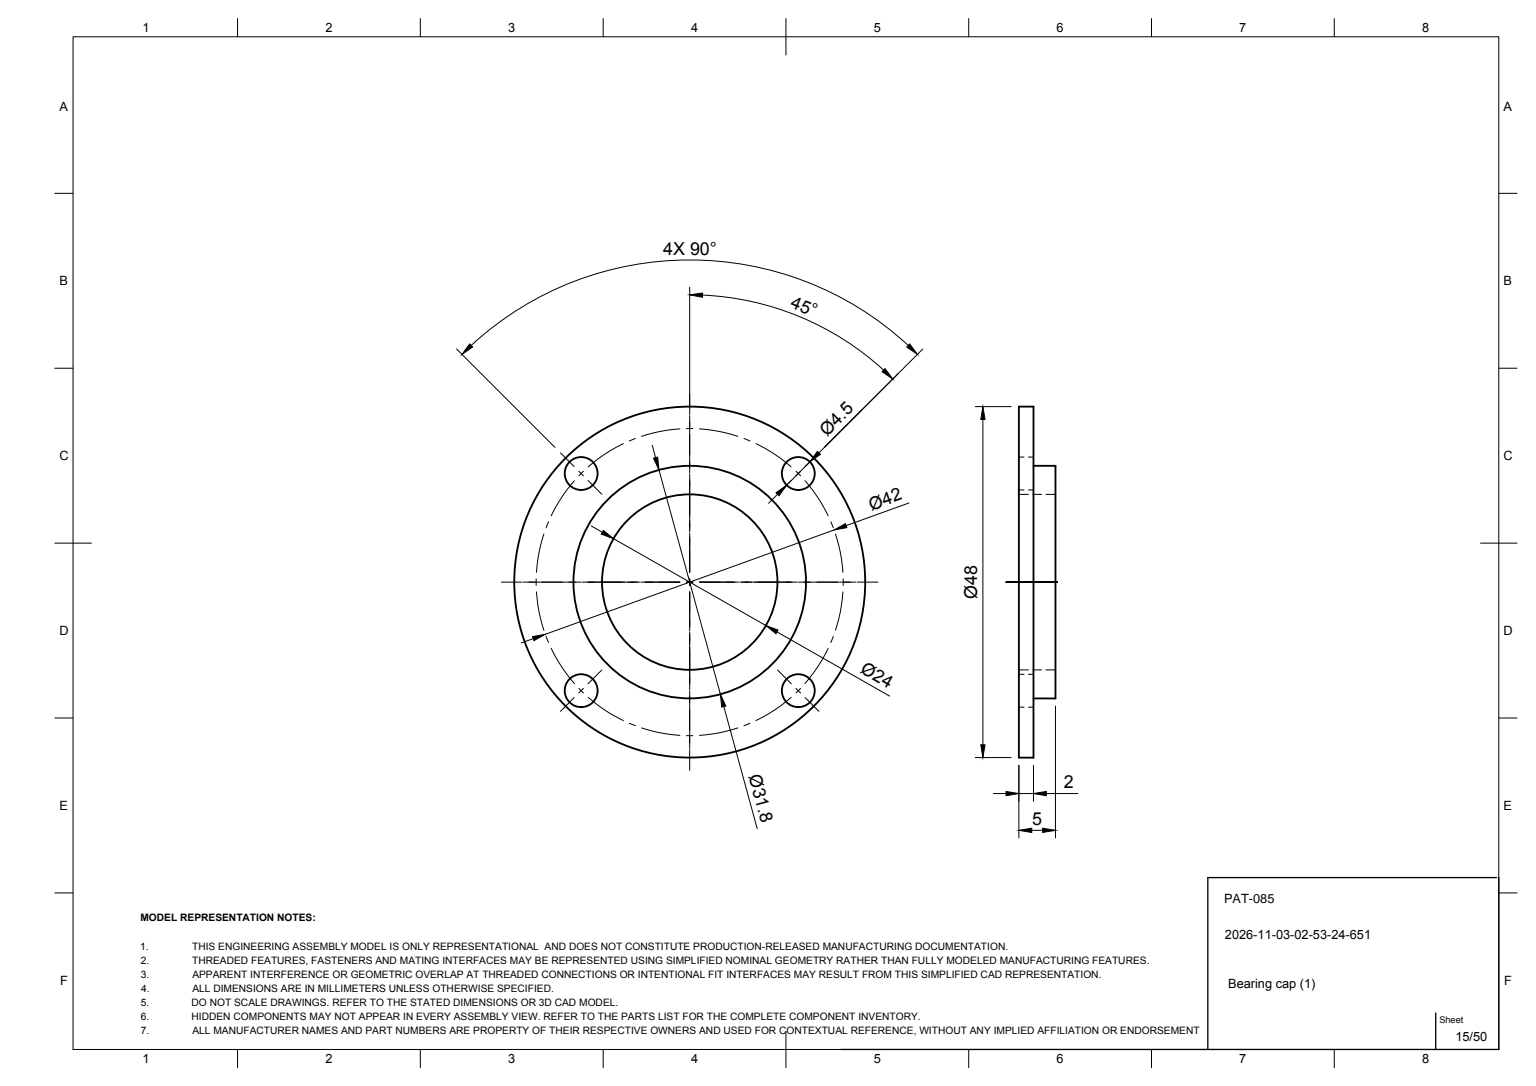
ISO-10303-21;
HEADER;
/* Generated by software containing ST-Developer
 * from STEP Tools, Inc. (www.steptools.com) 
 */

FILE_DESCRIPTION(
/* description */ ('Rack and pinion manual slide'),
/* implementation_level */ '2;1');

FILE_NAME(
/* name */ 'Bearing cap (1).step',
/* time_stamp */ '2026-10-28T03:22:49-07:00',
/* author */ (''),
/* organization */ (''),
/* preprocessor_version */ 'ST-DEVELOPER v20.2',
/* originating_system */ 'Autodesk Translation Framework v15.17.0.0',
/* authorisation */ '');

FILE_SCHEMA (('AUTOMOTIVE_DESIGN { 1 0 10303 214 3 1 1 }'));
ENDSEC;

DATA;
#10=MECHANICAL_DESIGN_GEOMETRIC_PRESENTATION_REPRESENTATION('',(#742),#34851);
#650=SHAPE_REPRESENTATION_RELATIONSHIP('SRR','None',#35085,#696);
#696=ADVANCED_BREP_SHAPE_REPRESENTATION('',(#795),#34810);
#742=STYLED_ITEM('',(#35411),#795);
#795=MANIFOLD_SOLID_BREP('Body1',#13762);
#910=FACE_BOUND('',#2464,.T.);
#911=FACE_BOUND('',#2468,.T.);
#912=FACE_BOUND('',#2469,.T.);
#913=FACE_BOUND('',#2470,.T.);
#914=FACE_BOUND('',#2471,.T.);
#915=FACE_BOUND('',#2472,.T.);
#916=FACE_BOUND('',#2474,.T.);
#917=FACE_BOUND('',#2475,.T.);
#918=FACE_BOUND('',#2476,.T.);
#919=FACE_BOUND('',#2477,.T.);
#920=FACE_BOUND('',#2478,.T.);
#1109=PLANE('',#14536);
#1110=PLANE('',#14543);
#1111=PLANE('',#14544);
#1642=FACE_OUTER_BOUND('',#2458,.T.);
#1643=FACE_OUTER_BOUND('',#2459,.T.);
#1644=FACE_OUTER_BOUND('',#2460,.T.);
#1645=FACE_OUTER_BOUND('',#2461,.T.);
#1646=FACE_OUTER_BOUND('',#2462,.T.);
#1647=FACE_OUTER_BOUND('',#2463,.T.);
#1648=FACE_OUTER_BOUND('',#2465,.T.);
#1649=FACE_OUTER_BOUND('',#2466,.T.);
#1650=FACE_OUTER_BOUND('',#2467,.T.);
#1651=FACE_OUTER_BOUND('',#2473,.T.);
#2458=EDGE_LOOP('',(#9726,#9727,#9728,#9729));
#2459=EDGE_LOOP('',(#9730,#9731,#9732,#9733));
#2460=EDGE_LOOP('',(#9734,#9735,#9736,#9737));
#2461=EDGE_LOOP('',(#9738,#9739,#9740,#9741));
#2462=EDGE_LOOP('',(#9742,#9743,#9744,#9745));
#2463=EDGE_LOOP('',(#9746));
#2464=EDGE_LOOP('',(#9747));
#2465=EDGE_LOOP('',(#9748,#9749,#9750,#9751));
#2466=EDGE_LOOP('',(#9752,#9753,#9754,#9755));
#2467=EDGE_LOOP('',(#9756));
#2468=EDGE_LOOP('',(#9757));
#2469=EDGE_LOOP('',(#9758));
#2470=EDGE_LOOP('',(#9759));
#2471=EDGE_LOOP('',(#9760));
#2472=EDGE_LOOP('',(#9761));
#2473=EDGE_LOOP('',(#9762));
#2474=EDGE_LOOP('',(#9763));
#2475=EDGE_LOOP('',(#9764));
#2476=EDGE_LOOP('',(#9765));
#2477=EDGE_LOOP('',(#9766));
#2478=EDGE_LOOP('',(#9767));
#3386=LINE('',#19991,#4677);
#3387=LINE('',#19997,#4678);
#3388=LINE('',#20003,#4679);
#3389=LINE('',#20009,#4680);
#3390=LINE('',#20015,#4681);
#3391=LINE('',#20023,#4682);
#3392=LINE('',#20028,#4683);
#4677=VECTOR('',#16174,0.225);
#4678=VECTOR('',#16181,0.225);
#4679=VECTOR('',#16188,0.225);
#4680=VECTOR('',#16195,0.225);
#4681=VECTOR('',#16202,1.59);
#4682=VECTOR('',#16213,1.2);
#4683=VECTOR('',#16218,2.4);
#5890=CIRCLE('',#14522,0.225);
#5891=CIRCLE('',#14523,0.225);
#5892=CIRCLE('',#14525,0.225);
#5893=CIRCLE('',#14526,0.225);
#5894=CIRCLE('',#14528,0.225);
#5895=CIRCLE('',#14529,0.225);
#5896=CIRCLE('',#14531,0.225);
#5897=CIRCLE('',#14532,0.225);
#5898=CIRCLE('',#14534,1.59);
#5899=CIRCLE('',#14535,1.59);
#5900=CIRCLE('',#14537,1.2);
#5901=CIRCLE('',#14539,1.2);
#5902=CIRCLE('',#14541,2.4);
#5903=CIRCLE('',#14542,2.4);
#6388=VERTEX_POINT('',#19988);
#6389=VERTEX_POINT('',#19990);
#6390=VERTEX_POINT('',#19994);
#6391=VERTEX_POINT('',#19996);
#6392=VERTEX_POINT('',#20000);
#6393=VERTEX_POINT('',#20002);
#6394=VERTEX_POINT('',#20006);
#6395=VERTEX_POINT('',#20008);
#6396=VERTEX_POINT('',#20012);
#6397=VERTEX_POINT('',#20014);
#6398=VERTEX_POINT('',#20018);
#6399=VERTEX_POINT('',#20021);
#6400=VERTEX_POINT('',#20025);
#6401=VERTEX_POINT('',#20027);
#7675=EDGE_CURVE('',#6388,#6388,#5890,.T.);
#7676=EDGE_CURVE('',#6388,#6389,#3386,.T.);
#7677=EDGE_CURVE('',#6389,#6389,#5891,.T.);
#7678=EDGE_CURVE('',#6390,#6390,#5892,.T.);
#7679=EDGE_CURVE('',#6390,#6391,#3387,.T.);
#7680=EDGE_CURVE('',#6391,#6391,#5893,.T.);
#7681=EDGE_CURVE('',#6392,#6392,#5894,.T.);
#7682=EDGE_CURVE('',#6392,#6393,#3388,.T.);
#7683=EDGE_CURVE('',#6393,#6393,#5895,.T.);
#7684=EDGE_CURVE('',#6394,#6394,#5896,.T.);
#7685=EDGE_CURVE('',#6394,#6395,#3389,.T.);
#7686=EDGE_CURVE('',#6395,#6395,#5897,.T.);
#7687=EDGE_CURVE('',#6396,#6396,#5898,.T.);
#7688=EDGE_CURVE('',#6396,#6397,#3390,.T.);
#7689=EDGE_CURVE('',#6397,#6397,#5899,.T.);
#7690=EDGE_CURVE('',#6398,#6398,#5900,.T.);
#7691=EDGE_CURVE('',#6399,#6399,#5901,.T.);
#7692=EDGE_CURVE('',#6399,#6398,#3391,.T.);
#7693=EDGE_CURVE('',#6400,#6400,#5902,.T.);
#7694=EDGE_CURVE('',#6400,#6401,#3392,.T.);
#7695=EDGE_CURVE('',#6401,#6401,#5903,.T.);
#9726=ORIENTED_EDGE('',*,*,#7675,.F.);
#9727=ORIENTED_EDGE('',*,*,#7676,.T.);
#9728=ORIENTED_EDGE('',*,*,#7677,.F.);
#9729=ORIENTED_EDGE('',*,*,#7676,.F.);
#9730=ORIENTED_EDGE('',*,*,#7678,.F.);
#9731=ORIENTED_EDGE('',*,*,#7679,.T.);
#9732=ORIENTED_EDGE('',*,*,#7680,.F.);
#9733=ORIENTED_EDGE('',*,*,#7679,.F.);
#9734=ORIENTED_EDGE('',*,*,#7681,.F.);
#9735=ORIENTED_EDGE('',*,*,#7682,.T.);
#9736=ORIENTED_EDGE('',*,*,#7683,.F.);
#9737=ORIENTED_EDGE('',*,*,#7682,.F.);
#9738=ORIENTED_EDGE('',*,*,#7684,.F.);
#9739=ORIENTED_EDGE('',*,*,#7685,.T.);
#9740=ORIENTED_EDGE('',*,*,#7686,.F.);
#9741=ORIENTED_EDGE('',*,*,#7685,.F.);
#9742=ORIENTED_EDGE('',*,*,#7687,.F.);
#9743=ORIENTED_EDGE('',*,*,#7688,.T.);
#9744=ORIENTED_EDGE('',*,*,#7689,.T.);
#9745=ORIENTED_EDGE('',*,*,#7688,.F.);
#9746=ORIENTED_EDGE('',*,*,#7689,.F.);
#9747=ORIENTED_EDGE('',*,*,#7690,.F.);
#9748=ORIENTED_EDGE('',*,*,#7691,.F.);
#9749=ORIENTED_EDGE('',*,*,#7692,.T.);
#9750=ORIENTED_EDGE('',*,*,#7690,.T.);
#9751=ORIENTED_EDGE('',*,*,#7692,.F.);
#9752=ORIENTED_EDGE('',*,*,#7693,.F.);
#9753=ORIENTED_EDGE('',*,*,#7694,.T.);
#9754=ORIENTED_EDGE('',*,*,#7695,.T.);
#9755=ORIENTED_EDGE('',*,*,#7694,.F.);
#9756=ORIENTED_EDGE('',*,*,#7693,.T.);
#9757=ORIENTED_EDGE('',*,*,#7691,.T.);
#9758=ORIENTED_EDGE('',*,*,#7686,.T.);
#9759=ORIENTED_EDGE('',*,*,#7683,.T.);
#9760=ORIENTED_EDGE('',*,*,#7680,.T.);
#9761=ORIENTED_EDGE('',*,*,#7677,.T.);
#9762=ORIENTED_EDGE('',*,*,#7695,.F.);
#9763=ORIENTED_EDGE('',*,*,#7687,.T.);
#9764=ORIENTED_EDGE('',*,*,#7684,.T.);
#9765=ORIENTED_EDGE('',*,*,#7681,.T.);
#9766=ORIENTED_EDGE('',*,*,#7678,.T.);
#9767=ORIENTED_EDGE('',*,*,#7675,.T.);
#12886=CYLINDRICAL_SURFACE('',#14521,0.225);
#12887=CYLINDRICAL_SURFACE('',#14524,0.225);
#12888=CYLINDRICAL_SURFACE('',#14527,0.225);
#12889=CYLINDRICAL_SURFACE('',#14530,0.225);
#12890=CYLINDRICAL_SURFACE('',#14533,1.59);
#12891=CYLINDRICAL_SURFACE('',#14538,1.2);
#12892=CYLINDRICAL_SURFACE('',#14540,2.4);
#13120=ADVANCED_FACE('',(#1642),#12886,.F.);
#13121=ADVANCED_FACE('',(#1643),#12887,.F.);
#13122=ADVANCED_FACE('',(#1644),#12888,.F.);
#13123=ADVANCED_FACE('',(#1645),#12889,.F.);
#13124=ADVANCED_FACE('',(#1646),#12890,.T.);
#13125=ADVANCED_FACE('',(#1647,#910),#1109,.F.);
#13126=ADVANCED_FACE('',(#1648),#12891,.F.);
#13127=ADVANCED_FACE('',(#1649),#12892,.T.);
#13128=ADVANCED_FACE('',(#1650,#911,#912,#913,#914,#915),#1110,.T.);
#13129=ADVANCED_FACE('',(#1651,#916,#917,#918,#919,#920),#1111,.F.);
#13762=CLOSED_SHELL('',(#13120,#13121,#13122,#13123,#13124,#13125,#13126,
#13127,#13128,#13129));
#14520=AXIS2_PLACEMENT_3D('',#19986,#16168,#16169);
#14521=AXIS2_PLACEMENT_3D('',#19987,#16170,#16171);
#14522=AXIS2_PLACEMENT_3D('',#19989,#16172,#16173);
#14523=AXIS2_PLACEMENT_3D('',#19992,#16175,#16176);
#14524=AXIS2_PLACEMENT_3D('',#19993,#16177,#16178);
#14525=AXIS2_PLACEMENT_3D('',#19995,#16179,#16180);
#14526=AXIS2_PLACEMENT_3D('',#19998,#16182,#16183);
#14527=AXIS2_PLACEMENT_3D('',#19999,#16184,#16185);
#14528=AXIS2_PLACEMENT_3D('',#20001,#16186,#16187);
#14529=AXIS2_PLACEMENT_3D('',#20004,#16189,#16190);
#14530=AXIS2_PLACEMENT_3D('',#20005,#16191,#16192);
#14531=AXIS2_PLACEMENT_3D('',#20007,#16193,#16194);
#14532=AXIS2_PLACEMENT_3D('',#20010,#16196,#16197);
#14533=AXIS2_PLACEMENT_3D('',#20011,#16198,#16199);
#14534=AXIS2_PLACEMENT_3D('',#20013,#16200,#16201);
#14535=AXIS2_PLACEMENT_3D('',#20016,#16203,#16204);
#14536=AXIS2_PLACEMENT_3D('',#20017,#16205,#16206);
#14537=AXIS2_PLACEMENT_3D('',#20019,#16207,#16208);
#14538=AXIS2_PLACEMENT_3D('',#20020,#16209,#16210);
#14539=AXIS2_PLACEMENT_3D('',#20022,#16211,#16212);
#14540=AXIS2_PLACEMENT_3D('',#20024,#16214,#16215);
#14541=AXIS2_PLACEMENT_3D('',#20026,#16216,#16217);
#14542=AXIS2_PLACEMENT_3D('',#20029,#16219,#16220);
#14543=AXIS2_PLACEMENT_3D('',#20030,#16221,#16222);
#14544=AXIS2_PLACEMENT_3D('',#20031,#16223,#16224);
#16168=DIRECTION('axis',(0.,0.,1.));
#16169=DIRECTION('refdir',(1.,0.,0.));
#16170=DIRECTION('center_axis',(0.,1.,0.));
#16171=DIRECTION('ref_axis',(1.,0.,0.));
#16172=DIRECTION('center_axis',(0.,1.,0.));
#16173=DIRECTION('ref_axis',(1.,0.,0.));
#16174=DIRECTION('',(0.,1.,0.));
#16175=DIRECTION('center_axis',(0.,-1.,0.));
#16176=DIRECTION('ref_axis',(1.,0.,0.));
#16177=DIRECTION('center_axis',(0.,1.,0.));
#16178=DIRECTION('ref_axis',(1.,0.,0.));
#16179=DIRECTION('center_axis',(0.,1.,0.));
#16180=DIRECTION('ref_axis',(1.,0.,0.));
#16181=DIRECTION('',(0.,1.,0.));
#16182=DIRECTION('center_axis',(0.,-1.,0.));
#16183=DIRECTION('ref_axis',(1.,0.,0.));
#16184=DIRECTION('center_axis',(0.,1.,0.));
#16185=DIRECTION('ref_axis',(1.,0.,0.));
#16186=DIRECTION('center_axis',(0.,1.,0.));
#16187=DIRECTION('ref_axis',(1.,0.,0.));
#16188=DIRECTION('',(0.,1.,0.));
#16189=DIRECTION('center_axis',(0.,-1.,0.));
#16190=DIRECTION('ref_axis',(1.,0.,0.));
#16191=DIRECTION('center_axis',(0.,1.,0.));
#16192=DIRECTION('ref_axis',(1.,0.,0.));
#16193=DIRECTION('center_axis',(0.,1.,0.));
#16194=DIRECTION('ref_axis',(1.,0.,0.));
#16195=DIRECTION('',(0.,1.,0.));
#16196=DIRECTION('center_axis',(0.,-1.,0.));
#16197=DIRECTION('ref_axis',(1.,0.,0.));
#16198=DIRECTION('center_axis',(0.,1.,0.));
#16199=DIRECTION('ref_axis',(1.,0.,0.));
#16200=DIRECTION('center_axis',(0.,1.,0.));
#16201=DIRECTION('ref_axis',(1.,0.,0.));
#16202=DIRECTION('',(0.,-1.,0.));
#16203=DIRECTION('center_axis',(0.,1.,0.));
#16204=DIRECTION('ref_axis',(1.,0.,0.));
#16205=DIRECTION('center_axis',(0.,1.,0.));
#16206=DIRECTION('ref_axis',(1.,0.,0.));
#16207=DIRECTION('center_axis',(0.,-1.,0.));
#16208=DIRECTION('ref_axis',(1.,0.,0.));
#16209=DIRECTION('center_axis',(0.,1.,0.));
#16210=DIRECTION('ref_axis',(1.,0.,0.));
#16211=DIRECTION('center_axis',(0.,-1.,0.));
#16212=DIRECTION('ref_axis',(1.,0.,0.));
#16213=DIRECTION('',(0.,-1.,0.));
#16214=DIRECTION('center_axis',(0.,1.,0.));
#16215=DIRECTION('ref_axis',(1.,0.,0.));
#16216=DIRECTION('center_axis',(0.,1.,0.));
#16217=DIRECTION('ref_axis',(1.,0.,0.));
#16218=DIRECTION('',(0.,-1.,0.));
#16219=DIRECTION('center_axis',(0.,1.,0.));
#16220=DIRECTION('ref_axis',(1.,0.,0.));
#16221=DIRECTION('center_axis',(0.,1.,0.));
#16222=DIRECTION('ref_axis',(1.,0.,0.));
#16223=DIRECTION('center_axis',(0.,1.,0.));
#16224=DIRECTION('ref_axis',(1.,0.,0.));
#19986=CARTESIAN_POINT('',(0.,0.,0.));
#19987=CARTESIAN_POINT('Origin',(9.51507575950825,-3.5,8.76507575950825));
#19988=CARTESIAN_POINT('',(9.29007575950825,-3.4,8.76507575950825));
#19989=CARTESIAN_POINT('Origin',(9.51507575950825,-3.4,8.76507575950825));
#19990=CARTESIAN_POINT('',(9.29007575950825,-3.2,8.76507575950825));
#19991=CARTESIAN_POINT('',(9.29007575950825,-3.5,8.76507575950825));
#19992=CARTESIAN_POINT('Origin',(9.51507575950825,-3.2,8.76507575950825));
#19993=CARTESIAN_POINT('Origin',(9.51507575950825,-3.5,11.7349242404918));
#19994=CARTESIAN_POINT('',(9.29007575950825,-3.4,11.7349242404918));
#19995=CARTESIAN_POINT('Origin',(9.51507575950825,-3.4,11.7349242404918));
#19996=CARTESIAN_POINT('',(9.29007575950825,-3.2,11.7349242404918));
#19997=CARTESIAN_POINT('',(9.29007575950825,-3.5,11.7349242404918));
#19998=CARTESIAN_POINT('Origin',(9.51507575950825,-3.2,11.7349242404918));
#19999=CARTESIAN_POINT('Origin',(12.4849242404918,-3.5,11.7349242404918));
#20000=CARTESIAN_POINT('',(12.2599242404918,-3.4,11.7349242404918));
#20001=CARTESIAN_POINT('Origin',(12.4849242404918,-3.4,11.7349242404918));
#20002=CARTESIAN_POINT('',(12.2599242404918,-3.2,11.7349242404918));
#20003=CARTESIAN_POINT('',(12.2599242404918,-3.5,11.7349242404918));
#20004=CARTESIAN_POINT('Origin',(12.4849242404918,-3.2,11.7349242404918));
#20005=CARTESIAN_POINT('Origin',(12.4849242404917,-3.5,8.76507575950825));
#20006=CARTESIAN_POINT('',(12.2599242404917,-3.4,8.76507575950825));
#20007=CARTESIAN_POINT('Origin',(12.4849242404917,-3.4,8.76507575950825));
#20008=CARTESIAN_POINT('',(12.2599242404917,-3.2,8.76507575950825));
#20009=CARTESIAN_POINT('',(12.2599242404917,-3.5,8.76507575950825));
#20010=CARTESIAN_POINT('Origin',(12.4849242404917,-3.2,8.76507575950825));
#20011=CARTESIAN_POINT('Origin',(11.,-3.7,10.25));
#20012=CARTESIAN_POINT('',(9.41,-3.4,10.25));
#20013=CARTESIAN_POINT('Origin',(11.,-3.4,10.25));
#20014=CARTESIAN_POINT('',(9.41,-3.7,10.25));
#20015=CARTESIAN_POINT('',(9.41,-3.7,10.25));
#20016=CARTESIAN_POINT('Origin',(11.,-3.7,10.25));
#20017=CARTESIAN_POINT('Origin',(11.,-3.7,10.25));
#20018=CARTESIAN_POINT('',(9.8,-3.7,10.25));
#20019=CARTESIAN_POINT('Origin',(11.,-3.7,10.25));
#20020=CARTESIAN_POINT('Origin',(11.,-3.4,10.25));
#20021=CARTESIAN_POINT('',(9.8,-3.2,10.25));
#20022=CARTESIAN_POINT('Origin',(11.,-3.2,10.25));
#20023=CARTESIAN_POINT('',(9.8,-3.4,10.25));
#20024=CARTESIAN_POINT('Origin',(11.,-3.4,10.25));
#20025=CARTESIAN_POINT('',(8.6,-3.2,10.25));
#20026=CARTESIAN_POINT('Origin',(11.,-3.2,10.25));
#20027=CARTESIAN_POINT('',(8.6,-3.4,10.25));
#20028=CARTESIAN_POINT('',(8.6,-3.4,10.25));
#20029=CARTESIAN_POINT('Origin',(11.,-3.4,10.25));
#20030=CARTESIAN_POINT('Origin',(11.,-3.2,10.25));
#20031=CARTESIAN_POINT('Origin',(11.,-3.4,10.25));
#34756=UNCERTAINTY_MEASURE_WITH_UNIT(LENGTH_MEASURE(0.001),#34852,
'DISTANCE_ACCURACY_VALUE',
'Maximum model space distance between geometric entities at asserted c
onnectivities');
#34797=UNCERTAINTY_MEASURE_WITH_UNIT(LENGTH_MEASURE(0.001),#34852,
'DISTANCE_ACCURACY_VALUE',
'Maximum model space distance between geometric entities at asserted c
onnectivities');
#34810=(
GEOMETRIC_REPRESENTATION_CONTEXT(3)
GLOBAL_UNCERTAINTY_ASSIGNED_CONTEXT((#34756))
GLOBAL_UNIT_ASSIGNED_CONTEXT((#34852,#34854,#34855))
REPRESENTATION_CONTEXT('','3D')
);
#34851=(
GEOMETRIC_REPRESENTATION_CONTEXT(3)
GLOBAL_UNCERTAINTY_ASSIGNED_CONTEXT((#34797))
GLOBAL_UNIT_ASSIGNED_CONTEXT((#34852,#34854,#34855))
REPRESENTATION_CONTEXT('','3D')
);
#34852=(
LENGTH_UNIT()
NAMED_UNIT(*)
SI_UNIT(.CENTI.,.METRE.)
);
#34854=(
NAMED_UNIT(*)
PLANE_ANGLE_UNIT()
SI_UNIT($,.RADIAN.)
);
#34855=(
NAMED_UNIT(*)
SI_UNIT($,.STERADIAN.)
SOLID_ANGLE_UNIT()
);
#34868=SHAPE_DEFINITION_REPRESENTATION(#34921,#35085);
#34921=PRODUCT_DEFINITION_SHAPE('',$,#35139);
#35085=SHAPE_REPRESENTATION('',(#14520),#34810);
#35126=PRODUCT_DEFINITION_CONTEXT('part definition',#35287,'design');
#35139=PRODUCT_DEFINITION('Bearing cap (1)','Bearing cap (1)',#35192,#35126);
#35192=PRODUCT_DEFINITION_FORMATION('',$,#35301);
#35287=APPLICATION_CONTEXT(
'Core Data for Automotive Mechanical Design Process');
#35288=PRODUCT_CONTEXT('part definition',#35287,'mechanical');
#35301=PRODUCT('Bearing cap (1)','Bearing cap (1)','Bearing cap (1)',(#35288));
#35405=COLOUR_RGB('Grey',0.48,0.52,0.57);
#35406=FILL_AREA_STYLE_COLOUR('',#35405);
#35407=FILL_AREA_STYLE('',(#35406));
#35408=SURFACE_STYLE_FILL_AREA(#35407);
#35409=SURFACE_SIDE_STYLE('',(#35408));
#35410=SURFACE_STYLE_USAGE(.BOTH.,#35409);
#35411=PRESENTATION_STYLE_ASSIGNMENT((#35410));
ENDSEC;
END-ISO-10303-21;
